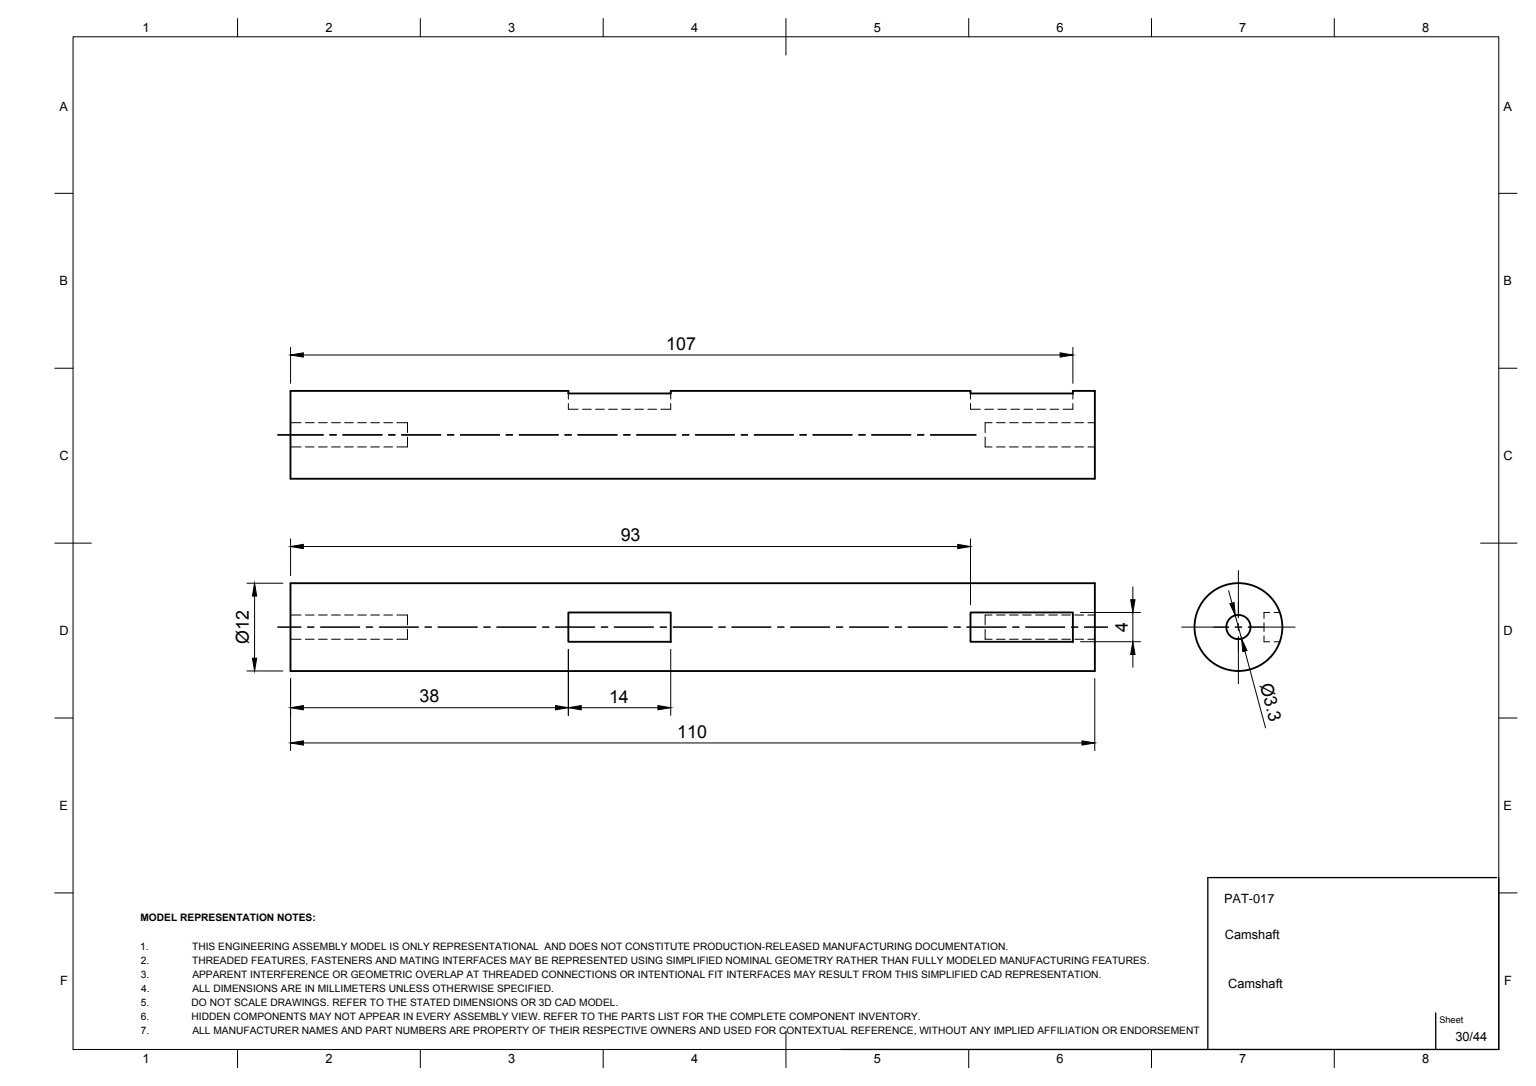
ISO-10303-21;
HEADER;
/* Generated by software containing ST-Developer
 * from STEP Tools, Inc. (www.steptools.com) 
 */

FILE_DESCRIPTION(
/* description */ ('Cam-and-follower valve demonstrator'),
/* implementation_level */ '2;1');

FILE_NAME(
/* name */ 'Camshaft.step',
/* time_stamp */ '2026-10-28T03:25:17-07:00',
/* author */ (''),
/* organization */ (''),
/* preprocessor_version */ 'ST-DEVELOPER v20.2',
/* originating_system */ 'Autodesk Translation Framework v15.17.0.0',
/* authorisation */ '');

FILE_SCHEMA (('AUTOMOTIVE_DESIGN { 1 0 10303 214 3 1 1 }'));
ENDSEC;

DATA;
#10=MECHANICAL_DESIGN_GEOMETRIC_PRESENTATION_REPRESENTATION('',(#440),#12896);
#361=SHAPE_REPRESENTATION_RELATIONSHIP('SRR','None',#13080,#397);
#397=ADVANCED_BREP_SHAPE_REPRESENTATION('',(#481),#12880);
#440=STYLED_ITEM('',(#13330),#481);
#481=MANIFOLD_SOLID_BREP('Body1',#6209);
#626=FACE_BOUND('',#1862,.T.);
#627=FACE_BOUND('',#1863,.T.);
#628=FACE_BOUND('',#1865,.T.);
#629=FACE_BOUND('',#1867,.T.);
#897=CIRCLE('',#7147,0.165);
#898=CIRCLE('',#7148,0.165);
#899=CIRCLE('',#7151,0.165);
#900=CIRCLE('',#7152,0.165);
#901=CIRCLE('',#7156,0.6);
#902=CIRCLE('',#7160,0.6);
#903=CIRCLE('',#7163,0.6);
#904=CIRCLE('',#7167,0.6);
#905=CIRCLE('',#7169,0.6);
#906=CIRCLE('',#7170,0.6);
#1062=CYLINDRICAL_SURFACE('',#7146,0.165);
#1063=CYLINDRICAL_SURFACE('',#7150,0.165);
#1064=CYLINDRICAL_SURFACE('',#7168,0.6);
#1348=FACE_OUTER_BOUND('',#1847,.T.);
#1349=FACE_OUTER_BOUND('',#1848,.T.);
#1350=FACE_OUTER_BOUND('',#1849,.T.);
#1351=FACE_OUTER_BOUND('',#1850,.T.);
#1352=FACE_OUTER_BOUND('',#1851,.T.);
#1353=FACE_OUTER_BOUND('',#1852,.T.);
#1354=FACE_OUTER_BOUND('',#1853,.T.);
#1355=FACE_OUTER_BOUND('',#1854,.T.);
#1356=FACE_OUTER_BOUND('',#1855,.T.);
#1357=FACE_OUTER_BOUND('',#1856,.T.);
#1358=FACE_OUTER_BOUND('',#1857,.T.);
#1359=FACE_OUTER_BOUND('',#1858,.T.);
#1360=FACE_OUTER_BOUND('',#1859,.T.);
#1361=FACE_OUTER_BOUND('',#1860,.T.);
#1362=FACE_OUTER_BOUND('',#1861,.T.);
#1363=FACE_OUTER_BOUND('',#1864,.T.);
#1364=FACE_OUTER_BOUND('',#1866,.T.);
#1847=EDGE_LOOP('',(#5173,#5174,#5175,#5176));
#1848=EDGE_LOOP('',(#5177));
#1849=EDGE_LOOP('',(#5178,#5179,#5180,#5181));
#1850=EDGE_LOOP('',(#5182));
#1851=EDGE_LOOP('',(#5183,#5184,#5185,#5186));
#1852=EDGE_LOOP('',(#5187,#5188,#5189,#5190));
#1853=EDGE_LOOP('',(#5191,#5192,#5193,#5194));
#1854=EDGE_LOOP('',(#5195,#5196,#5197,#5198));
#1855=EDGE_LOOP('',(#5199,#5200,#5201,#5202));
#1856=EDGE_LOOP('',(#5203,#5204,#5205,#5206));
#1857=EDGE_LOOP('',(#5207,#5208,#5209,#5210));
#1858=EDGE_LOOP('',(#5211,#5212,#5213,#5214));
#1859=EDGE_LOOP('',(#5215,#5216,#5217,#5218));
#1860=EDGE_LOOP('',(#5219,#5220,#5221,#5222));
#1861=EDGE_LOOP('',(#5223,#5224,#5225,#5226));
#1862=EDGE_LOOP('',(#5227,#5228,#5229,#5230));
#1863=EDGE_LOOP('',(#5231,#5232,#5233,#5234));
#1864=EDGE_LOOP('',(#5235));
#1865=EDGE_LOOP('',(#5236));
#1866=EDGE_LOOP('',(#5237));
#1867=EDGE_LOOP('',(#5238));
#2281=LINE('',#12271,#2703);
#2282=LINE('',#12278,#2704);
#2283=LINE('',#12284,#2705);
#2284=LINE('',#12286,#2706);
#2285=LINE('',#12288,#2707);
#2286=LINE('',#12289,#2708);
#2287=LINE('',#12294,#2709);
#2288=LINE('',#12295,#2710);
#2289=LINE('',#12298,#2711);
#2290=LINE('',#12300,#2712);
#2291=LINE('',#12301,#2713);
#2292=LINE('',#12303,#2714);
#2293=LINE('',#12309,#2715);
#2294=LINE('',#12311,#2716);
#2295=LINE('',#12313,#2717);
#2296=LINE('',#12314,#2718);
#2297=LINE('',#12319,#2719);
#2298=LINE('',#12320,#2720);
#2299=LINE('',#12323,#2721);
#2300=LINE('',#12325,#2722);
#2301=LINE('',#12326,#2723);
#2302=LINE('',#12328,#2724);
#2303=LINE('',#12335,#2725);
#2703=VECTOR('',#8752,0.165);
#2704=VECTOR('',#8761,0.165);
#2705=VECTOR('',#8768,1.);
#2706=VECTOR('',#8769,1.);
#2707=VECTOR('',#8770,1.);
#2708=VECTOR('',#8771,1.);
#2709=VECTOR('',#8776,1.);
#2710=VECTOR('',#8777,1.);
#2711=VECTOR('',#8780,1.);
#2712=VECTOR('',#8781,1.);
#2713=VECTOR('',#8782,1.);
#2714=VECTOR('',#8785,1.);
#2715=VECTOR('',#8792,1.);
#2716=VECTOR('',#8793,1.);
#2717=VECTOR('',#8794,1.);
#2718=VECTOR('',#8795,1.);
#2719=VECTOR('',#8800,1.);
#2720=VECTOR('',#8801,1.);
#2721=VECTOR('',#8804,1.);
#2722=VECTOR('',#8805,1.);
#2723=VECTOR('',#8806,1.);
#2724=VECTOR('',#8809,1.);
#2725=VECTOR('',#8818,0.6);
#3204=VERTEX_POINT('',#12268);
#3205=VERTEX_POINT('',#12270);
#3206=VERTEX_POINT('',#12275);
#3207=VERTEX_POINT('',#12277);
#3208=VERTEX_POINT('',#12282);
#3209=VERTEX_POINT('',#12283);
#3210=VERTEX_POINT('',#12285);
#3211=VERTEX_POINT('',#12287);
#3212=VERTEX_POINT('',#12291);
#3213=VERTEX_POINT('',#12293);
#3214=VERTEX_POINT('',#12297);
#3215=VERTEX_POINT('',#12299);
#3216=VERTEX_POINT('',#12307);
#3217=VERTEX_POINT('',#12308);
#3218=VERTEX_POINT('',#12310);
#3219=VERTEX_POINT('',#12312);
#3220=VERTEX_POINT('',#12316);
#3221=VERTEX_POINT('',#12318);
#3222=VERTEX_POINT('',#12322);
#3223=VERTEX_POINT('',#12324);
#3224=VERTEX_POINT('',#12332);
#3225=VERTEX_POINT('',#12334);
#3883=EDGE_CURVE('',#3204,#3204,#897,.T.);
#3884=EDGE_CURVE('',#3204,#3205,#2281,.T.);
#3885=EDGE_CURVE('',#3205,#3205,#898,.T.);
#3886=EDGE_CURVE('',#3206,#3206,#899,.T.);
#3887=EDGE_CURVE('',#3206,#3207,#2282,.T.);
#3888=EDGE_CURVE('',#3207,#3207,#900,.T.);
#3889=EDGE_CURVE('',#3208,#3209,#2283,.T.);
#3890=EDGE_CURVE('',#3208,#3210,#2284,.T.);
#3891=EDGE_CURVE('',#3211,#3210,#2285,.T.);
#3892=EDGE_CURVE('',#3211,#3209,#2286,.T.);
#3893=EDGE_CURVE('',#3209,#3212,#901,.T.);
#3894=EDGE_CURVE('',#3213,#3211,#2287,.T.);
#3895=EDGE_CURVE('',#3212,#3213,#2288,.T.);
#3896=EDGE_CURVE('',#3212,#3214,#2289,.T.);
#3897=EDGE_CURVE('',#3213,#3215,#2290,.T.);
#3898=EDGE_CURVE('',#3215,#3214,#2291,.T.);
#3899=EDGE_CURVE('',#3210,#3215,#2292,.T.);
#3900=EDGE_CURVE('',#3214,#3208,#902,.T.);
#3901=EDGE_CURVE('',#3216,#3217,#2293,.T.);
#3902=EDGE_CURVE('',#3216,#3218,#2294,.T.);
#3903=EDGE_CURVE('',#3219,#3218,#2295,.T.);
#3904=EDGE_CURVE('',#3219,#3217,#2296,.T.);
#3905=EDGE_CURVE('',#3217,#3220,#903,.T.);
#3906=EDGE_CURVE('',#3221,#3219,#2297,.T.);
#3907=EDGE_CURVE('',#3220,#3221,#2298,.T.);
#3908=EDGE_CURVE('',#3220,#3222,#2299,.T.);
#3909=EDGE_CURVE('',#3221,#3223,#2300,.T.);
#3910=EDGE_CURVE('',#3223,#3222,#2301,.T.);
#3911=EDGE_CURVE('',#3218,#3223,#2302,.T.);
#3912=EDGE_CURVE('',#3222,#3216,#904,.T.);
#3913=EDGE_CURVE('',#3224,#3224,#905,.T.);
#3914=EDGE_CURVE('',#3224,#3225,#2303,.T.);
#3915=EDGE_CURVE('',#3225,#3225,#906,.T.);
#5173=ORIENTED_EDGE('',*,*,#3883,.F.);
#5174=ORIENTED_EDGE('',*,*,#3884,.T.);
#5175=ORIENTED_EDGE('',*,*,#3885,.F.);
#5176=ORIENTED_EDGE('',*,*,#3884,.F.);
#5177=ORIENTED_EDGE('',*,*,#3883,.T.);
#5178=ORIENTED_EDGE('',*,*,#3886,.F.);
#5179=ORIENTED_EDGE('',*,*,#3887,.T.);
#5180=ORIENTED_EDGE('',*,*,#3888,.T.);
#5181=ORIENTED_EDGE('',*,*,#3887,.F.);
#5182=ORIENTED_EDGE('',*,*,#3888,.F.);
#5183=ORIENTED_EDGE('',*,*,#3889,.F.);
#5184=ORIENTED_EDGE('',*,*,#3890,.T.);
#5185=ORIENTED_EDGE('',*,*,#3891,.F.);
#5186=ORIENTED_EDGE('',*,*,#3892,.T.);
#5187=ORIENTED_EDGE('',*,*,#3893,.F.);
#5188=ORIENTED_EDGE('',*,*,#3892,.F.);
#5189=ORIENTED_EDGE('',*,*,#3894,.F.);
#5190=ORIENTED_EDGE('',*,*,#3895,.F.);
#5191=ORIENTED_EDGE('',*,*,#3896,.F.);
#5192=ORIENTED_EDGE('',*,*,#3895,.T.);
#5193=ORIENTED_EDGE('',*,*,#3897,.T.);
#5194=ORIENTED_EDGE('',*,*,#3898,.T.);
#5195=ORIENTED_EDGE('',*,*,#3894,.T.);
#5196=ORIENTED_EDGE('',*,*,#3891,.T.);
#5197=ORIENTED_EDGE('',*,*,#3899,.T.);
#5198=ORIENTED_EDGE('',*,*,#3897,.F.);
#5199=ORIENTED_EDGE('',*,*,#3900,.F.);
#5200=ORIENTED_EDGE('',*,*,#3898,.F.);
#5201=ORIENTED_EDGE('',*,*,#3899,.F.);
#5202=ORIENTED_EDGE('',*,*,#3890,.F.);
#5203=ORIENTED_EDGE('',*,*,#3901,.F.);
#5204=ORIENTED_EDGE('',*,*,#3902,.T.);
#5205=ORIENTED_EDGE('',*,*,#3903,.F.);
#5206=ORIENTED_EDGE('',*,*,#3904,.T.);
#5207=ORIENTED_EDGE('',*,*,#3905,.F.);
#5208=ORIENTED_EDGE('',*,*,#3904,.F.);
#5209=ORIENTED_EDGE('',*,*,#3906,.F.);
#5210=ORIENTED_EDGE('',*,*,#3907,.F.);
#5211=ORIENTED_EDGE('',*,*,#3908,.F.);
#5212=ORIENTED_EDGE('',*,*,#3907,.T.);
#5213=ORIENTED_EDGE('',*,*,#3909,.T.);
#5214=ORIENTED_EDGE('',*,*,#3910,.T.);
#5215=ORIENTED_EDGE('',*,*,#3906,.T.);
#5216=ORIENTED_EDGE('',*,*,#3903,.T.);
#5217=ORIENTED_EDGE('',*,*,#3911,.T.);
#5218=ORIENTED_EDGE('',*,*,#3909,.F.);
#5219=ORIENTED_EDGE('',*,*,#3912,.F.);
#5220=ORIENTED_EDGE('',*,*,#3910,.F.);
#5221=ORIENTED_EDGE('',*,*,#3911,.F.);
#5222=ORIENTED_EDGE('',*,*,#3902,.F.);
#5223=ORIENTED_EDGE('',*,*,#3913,.F.);
#5224=ORIENTED_EDGE('',*,*,#3914,.T.);
#5225=ORIENTED_EDGE('',*,*,#3915,.T.);
#5226=ORIENTED_EDGE('',*,*,#3914,.F.);
#5227=ORIENTED_EDGE('',*,*,#3896,.T.);
#5228=ORIENTED_EDGE('',*,*,#3900,.T.);
#5229=ORIENTED_EDGE('',*,*,#3889,.T.);
#5230=ORIENTED_EDGE('',*,*,#3893,.T.);
#5231=ORIENTED_EDGE('',*,*,#3908,.T.);
#5232=ORIENTED_EDGE('',*,*,#3912,.T.);
#5233=ORIENTED_EDGE('',*,*,#3901,.T.);
#5234=ORIENTED_EDGE('',*,*,#3905,.T.);
#5235=ORIENTED_EDGE('',*,*,#3913,.T.);
#5236=ORIENTED_EDGE('',*,*,#3885,.T.);
#5237=ORIENTED_EDGE('',*,*,#3915,.F.);
#5238=ORIENTED_EDGE('',*,*,#3886,.T.);
#5733=PLANE('',#7149);
#5734=PLANE('',#7153);
#5735=PLANE('',#7154);
#5736=PLANE('',#7155);
#5737=PLANE('',#7157);
#5738=PLANE('',#7158);
#5739=PLANE('',#7159);
#5740=PLANE('',#7161);
#5741=PLANE('',#7162);
#5742=PLANE('',#7164);
#5743=PLANE('',#7165);
#5744=PLANE('',#7166);
#5745=PLANE('',#7171);
#5746=PLANE('',#7172);
#6064=ADVANCED_FACE('',(#1348),#1062,.F.);
#6065=ADVANCED_FACE('',(#1349),#5733,.T.);
#6066=ADVANCED_FACE('',(#1350),#1063,.F.);
#6067=ADVANCED_FACE('',(#1351),#5734,.F.);
#6068=ADVANCED_FACE('',(#1352),#5735,.F.);
#6069=ADVANCED_FACE('',(#1353),#5736,.T.);
#6070=ADVANCED_FACE('',(#1354),#5737,.F.);
#6071=ADVANCED_FACE('',(#1355),#5738,.F.);
#6072=ADVANCED_FACE('',(#1356),#5739,.F.);
#6073=ADVANCED_FACE('',(#1357),#5740,.F.);
#6074=ADVANCED_FACE('',(#1358),#5741,.T.);
#6075=ADVANCED_FACE('',(#1359),#5742,.F.);
#6076=ADVANCED_FACE('',(#1360),#5743,.F.);
#6077=ADVANCED_FACE('',(#1361),#5744,.F.);
#6078=ADVANCED_FACE('',(#1362,#626,#627),#1064,.T.);
#6079=ADVANCED_FACE('',(#1363,#628),#5745,.T.);
#6080=ADVANCED_FACE('',(#1364,#629),#5746,.F.);
#6209=CLOSED_SHELL('',(#6064,#6065,#6066,#6067,#6068,#6069,#6070,#6071,
#6072,#6073,#6074,#6075,#6076,#6077,#6078,#6079,#6080));
#7145=AXIS2_PLACEMENT_3D('',#12266,#8746,#8747);
#7146=AXIS2_PLACEMENT_3D('',#12267,#8748,#8749);
#7147=AXIS2_PLACEMENT_3D('',#12269,#8750,#8751);
#7148=AXIS2_PLACEMENT_3D('',#12272,#8753,#8754);
#7149=AXIS2_PLACEMENT_3D('',#12273,#8755,#8756);
#7150=AXIS2_PLACEMENT_3D('',#12274,#8757,#8758);
#7151=AXIS2_PLACEMENT_3D('',#12276,#8759,#8760);
#7152=AXIS2_PLACEMENT_3D('',#12279,#8762,#8763);
#7153=AXIS2_PLACEMENT_3D('',#12280,#8764,#8765);
#7154=AXIS2_PLACEMENT_3D('',#12281,#8766,#8767);
#7155=AXIS2_PLACEMENT_3D('',#12290,#8772,#8773);
#7156=AXIS2_PLACEMENT_3D('',#12292,#8774,#8775);
#7157=AXIS2_PLACEMENT_3D('',#12296,#8778,#8779);
#7158=AXIS2_PLACEMENT_3D('',#12302,#8783,#8784);
#7159=AXIS2_PLACEMENT_3D('',#12304,#8786,#8787);
#7160=AXIS2_PLACEMENT_3D('',#12305,#8788,#8789);
#7161=AXIS2_PLACEMENT_3D('',#12306,#8790,#8791);
#7162=AXIS2_PLACEMENT_3D('',#12315,#8796,#8797);
#7163=AXIS2_PLACEMENT_3D('',#12317,#8798,#8799);
#7164=AXIS2_PLACEMENT_3D('',#12321,#8802,#8803);
#7165=AXIS2_PLACEMENT_3D('',#12327,#8807,#8808);
#7166=AXIS2_PLACEMENT_3D('',#12329,#8810,#8811);
#7167=AXIS2_PLACEMENT_3D('',#12330,#8812,#8813);
#7168=AXIS2_PLACEMENT_3D('',#12331,#8814,#8815);
#7169=AXIS2_PLACEMENT_3D('',#12333,#8816,#8817);
#7170=AXIS2_PLACEMENT_3D('',#12336,#8819,#8820);
#7171=AXIS2_PLACEMENT_3D('',#12337,#8821,#8822);
#7172=AXIS2_PLACEMENT_3D('',#12338,#8823,#8824);
#8746=DIRECTION('axis',(0.,0.,1.));
#8747=DIRECTION('refdir',(1.,0.,0.));
#8748=DIRECTION('center_axis',(0.,1.,0.));
#8749=DIRECTION('ref_axis',(1.,0.,0.));
#8750=DIRECTION('center_axis',(0.,1.,0.));
#8751=DIRECTION('ref_axis',(1.,0.,0.));
#8752=DIRECTION('',(0.,1.,0.));
#8753=DIRECTION('center_axis',(0.,-1.,0.));
#8754=DIRECTION('ref_axis',(1.,0.,0.));
#8755=DIRECTION('center_axis',(0.,1.,0.));
#8756=DIRECTION('ref_axis',(1.,0.,0.));
#8757=DIRECTION('center_axis',(0.,1.,0.));
#8758=DIRECTION('ref_axis',(1.,0.,0.));
#8759=DIRECTION('center_axis',(0.,1.,0.));
#8760=DIRECTION('ref_axis',(1.,0.,0.));
#8761=DIRECTION('',(0.,1.,0.));
#8762=DIRECTION('center_axis',(0.,1.,0.));
#8763=DIRECTION('ref_axis',(1.,0.,0.));
#8764=DIRECTION('center_axis',(0.,1.,0.));
#8765=DIRECTION('ref_axis',(1.,0.,0.));
#8766=DIRECTION('center_axis',(-1.,0.,0.));
#8767=DIRECTION('ref_axis',(0.,0.,1.));
#8768=DIRECTION('',(0.,-1.,0.));
#8769=DIRECTION('',(0.,0.,1.));
#8770=DIRECTION('',(0.,1.,0.));
#8771=DIRECTION('',(0.,0.,-1.));
#8772=DIRECTION('center_axis',(0.,1.,0.));
#8773=DIRECTION('ref_axis',(1.,0.,0.));
#8774=DIRECTION('center_axis',(0.,-1.,0.));
#8775=DIRECTION('ref_axis',(1.,0.,0.));
#8776=DIRECTION('',(-1.,0.,0.));
#8777=DIRECTION('',(0.,0.,1.));
#8778=DIRECTION('center_axis',(1.,0.,0.));
#8779=DIRECTION('ref_axis',(0.,0.,-1.));
#8780=DIRECTION('',(0.,1.,0.));
#8781=DIRECTION('',(0.,1.,0.));
#8782=DIRECTION('',(0.,0.,-1.));
#8783=DIRECTION('center_axis',(0.,0.,1.));
#8784=DIRECTION('ref_axis',(1.,0.,0.));
#8785=DIRECTION('',(1.,0.,0.));
#8786=DIRECTION('center_axis',(0.,1.,0.));
#8787=DIRECTION('ref_axis',(0.,0.,1.));
#8788=DIRECTION('center_axis',(0.,1.,0.));
#8789=DIRECTION('ref_axis',(1.,0.,0.));
#8790=DIRECTION('center_axis',(-1.,0.,0.));
#8791=DIRECTION('ref_axis',(0.,0.,1.));
#8792=DIRECTION('',(0.,-1.,0.));
#8793=DIRECTION('',(0.,0.,1.));
#8794=DIRECTION('',(0.,1.,0.));
#8795=DIRECTION('',(0.,0.,-1.));
#8796=DIRECTION('center_axis',(0.,1.,0.));
#8797=DIRECTION('ref_axis',(1.,0.,0.));
#8798=DIRECTION('center_axis',(0.,-1.,0.));
#8799=DIRECTION('ref_axis',(1.,0.,0.));
#8800=DIRECTION('',(-1.,0.,0.));
#8801=DIRECTION('',(0.,0.,1.));
#8802=DIRECTION('center_axis',(1.,0.,0.));
#8803=DIRECTION('ref_axis',(0.,0.,-1.));
#8804=DIRECTION('',(0.,1.,0.));
#8805=DIRECTION('',(0.,1.,0.));
#8806=DIRECTION('',(0.,0.,-1.));
#8807=DIRECTION('center_axis',(0.,0.,1.));
#8808=DIRECTION('ref_axis',(1.,0.,0.));
#8809=DIRECTION('',(1.,0.,0.));
#8810=DIRECTION('center_axis',(0.,1.,0.));
#8811=DIRECTION('ref_axis',(0.,0.,1.));
#8812=DIRECTION('center_axis',(0.,1.,0.));
#8813=DIRECTION('ref_axis',(1.,0.,0.));
#8814=DIRECTION('center_axis',(0.,1.,0.));
#8815=DIRECTION('ref_axis',(1.,0.,0.));
#8816=DIRECTION('center_axis',(0.,1.,0.));
#8817=DIRECTION('ref_axis',(1.,0.,0.));
#8818=DIRECTION('',(0.,-1.,0.));
#8819=DIRECTION('center_axis',(0.,1.,0.));
#8820=DIRECTION('ref_axis',(1.,0.,0.));
#8821=DIRECTION('center_axis',(0.,1.,0.));
#8822=DIRECTION('ref_axis',(1.,0.,0.));
#8823=DIRECTION('center_axis',(0.,1.,0.));
#8824=DIRECTION('ref_axis',(1.,0.,0.));
#12266=CARTESIAN_POINT('',(0.,0.,0.));
#12267=CARTESIAN_POINT('Origin',(0.,5.,4.));
#12268=CARTESIAN_POINT('',(-0.165,5.,4.));
#12269=CARTESIAN_POINT('Origin',(0.,5.,4.));
#12270=CARTESIAN_POINT('',(-0.165,6.5,4.));
#12271=CARTESIAN_POINT('',(-0.165,5.,4.));
#12272=CARTESIAN_POINT('Origin',(0.,6.5,4.));
#12273=CARTESIAN_POINT('Origin',(0.,5.,4.));
#12274=CARTESIAN_POINT('Origin',(0.,-4.6,4.));
#12275=CARTESIAN_POINT('',(-0.165,-4.5,4.));
#12276=CARTESIAN_POINT('Origin',(0.,-4.5,4.));
#12277=CARTESIAN_POINT('',(-0.165,-2.9,4.));
#12278=CARTESIAN_POINT('',(-0.165,-4.6,4.));
#12279=CARTESIAN_POINT('Origin',(0.,-2.9,4.));
#12280=CARTESIAN_POINT('Origin',(0.,-2.9,4.));
#12281=CARTESIAN_POINT('Origin',(-0.2,4.8,3.3));
#12282=CARTESIAN_POINT('',(-0.2,6.2,3.43431457505076));
#12283=CARTESIAN_POINT('',(-0.2,4.8,3.43431457505076));
#12284=CARTESIAN_POINT('',(-0.2,-4.5,3.43431457505076));
#12285=CARTESIAN_POINT('',(-0.2,6.2,3.65));
#12286=CARTESIAN_POINT('',(-0.2,6.2,3.65));
#12287=CARTESIAN_POINT('',(-0.2,4.8,3.65));
#12288=CARTESIAN_POINT('',(-0.2,4.8,3.65));
#12289=CARTESIAN_POINT('',(-0.2,4.8,3.65));
#12290=CARTESIAN_POINT('Origin',(0.,4.8,3.475));
#12291=CARTESIAN_POINT('',(0.2,4.8,3.43431457505076));
#12292=CARTESIAN_POINT('Origin',(0.,4.8,4.));
#12293=CARTESIAN_POINT('',(0.2,4.8,3.65));
#12294=CARTESIAN_POINT('',(0.2,4.8,3.65));
#12295=CARTESIAN_POINT('',(0.2,4.8,3.3));
#12296=CARTESIAN_POINT('Origin',(0.2,4.8,3.65));
#12297=CARTESIAN_POINT('',(0.2,6.2,3.43431457505076));
#12298=CARTESIAN_POINT('',(0.2,-4.5,3.43431457505076));
#12299=CARTESIAN_POINT('',(0.2,6.2,3.65));
#12300=CARTESIAN_POINT('',(0.2,4.8,3.65));
#12301=CARTESIAN_POINT('',(0.2,6.2,3.3));
#12302=CARTESIAN_POINT('Origin',(-0.2,4.8,3.65));
#12303=CARTESIAN_POINT('',(0.2,6.2,3.65));
#12304=CARTESIAN_POINT('Origin',(0.,6.2,3.475));
#12305=CARTESIAN_POINT('Origin',(0.,6.2,4.));
#12306=CARTESIAN_POINT('Origin',(-0.2,-0.7,3.3));
#12307=CARTESIAN_POINT('',(-0.2,0.7,3.43431457505076));
#12308=CARTESIAN_POINT('',(-0.2,-0.7,3.43431457505076));
#12309=CARTESIAN_POINT('',(-0.2,-4.5,3.43431457505076));
#12310=CARTESIAN_POINT('',(-0.2,0.7,3.65));
#12311=CARTESIAN_POINT('',(-0.2,0.7,3.65));
#12312=CARTESIAN_POINT('',(-0.2,-0.7,3.65));
#12313=CARTESIAN_POINT('',(-0.2,-0.7,3.65));
#12314=CARTESIAN_POINT('',(-0.2,-0.7,3.65));
#12315=CARTESIAN_POINT('Origin',(0.,-0.7,3.475));
#12316=CARTESIAN_POINT('',(0.2,-0.7,3.43431457505076));
#12317=CARTESIAN_POINT('Origin',(0.,-0.7,4.));
#12318=CARTESIAN_POINT('',(0.2,-0.7,3.65));
#12319=CARTESIAN_POINT('',(0.2,-0.7,3.65));
#12320=CARTESIAN_POINT('',(0.2,-0.7,3.3));
#12321=CARTESIAN_POINT('Origin',(0.2,-0.7,3.65));
#12322=CARTESIAN_POINT('',(0.2,0.7,3.43431457505076));
#12323=CARTESIAN_POINT('',(0.2,-4.5,3.43431457505076));
#12324=CARTESIAN_POINT('',(0.2,0.7,3.65));
#12325=CARTESIAN_POINT('',(0.2,-0.7,3.65));
#12326=CARTESIAN_POINT('',(0.2,0.7,3.3));
#12327=CARTESIAN_POINT('Origin',(-0.2,-0.7,3.65));
#12328=CARTESIAN_POINT('',(0.2,0.7,3.65));
#12329=CARTESIAN_POINT('Origin',(0.,0.7,3.475));
#12330=CARTESIAN_POINT('Origin',(0.,0.7,4.));
#12331=CARTESIAN_POINT('Origin',(0.,-4.5,4.));
#12332=CARTESIAN_POINT('',(-0.6,6.5,4.));
#12333=CARTESIAN_POINT('Origin',(0.,6.5,4.));
#12334=CARTESIAN_POINT('',(-0.6,-4.5,4.));
#12335=CARTESIAN_POINT('',(-0.6,-4.5,4.));
#12336=CARTESIAN_POINT('Origin',(0.,-4.5,4.));
#12337=CARTESIAN_POINT('Origin',(0.,6.5,4.));
#12338=CARTESIAN_POINT('Origin',(0.,-4.5,4.));
#12837=UNCERTAINTY_MEASURE_WITH_UNIT(LENGTH_MEASURE(0.001),#12897,
'DISTANCE_ACCURACY_VALUE',
'Maximum model space distance between geometric entities at asserted c
onnectivities');
#12853=UNCERTAINTY_MEASURE_WITH_UNIT(LENGTH_MEASURE(0.001),#12897,
'DISTANCE_ACCURACY_VALUE',
'Maximum model space distance between geometric entities at asserted c
onnectivities');
#12880=(
GEOMETRIC_REPRESENTATION_CONTEXT(3)
GLOBAL_UNCERTAINTY_ASSIGNED_CONTEXT((#12837))
GLOBAL_UNIT_ASSIGNED_CONTEXT((#12897,#12899,#12900))
REPRESENTATION_CONTEXT('','3D')
);
#12896=(
GEOMETRIC_REPRESENTATION_CONTEXT(3)
GLOBAL_UNCERTAINTY_ASSIGNED_CONTEXT((#12853))
GLOBAL_UNIT_ASSIGNED_CONTEXT((#12897,#12899,#12900))
REPRESENTATION_CONTEXT('','3D')
);
#12897=(
LENGTH_UNIT()
NAMED_UNIT(*)
SI_UNIT(.CENTI.,.METRE.)
);
#12899=(
NAMED_UNIT(*)
PLANE_ANGLE_UNIT()
SI_UNIT($,.RADIAN.)
);
#12900=(
NAMED_UNIT(*)
SI_UNIT($,.STERADIAN.)
SOLID_ANGLE_UNIT()
);
#12927=SHAPE_DEFINITION_REPRESENTATION(#12976,#13080);
#12976=PRODUCT_DEFINITION_SHAPE('',$,#13123);
#13080=SHAPE_REPRESENTATION('',(#7145),#12880);
#13096=PRODUCT_DEFINITION_CONTEXT('part definition',#13224,'design');
#13123=PRODUCT_DEFINITION('Camshaft','Camshaft',#13165,#13096);
#13165=PRODUCT_DEFINITION_FORMATION('',$,#13252);
#13224=APPLICATION_CONTEXT(
'Core Data for Automotive Mechanical Design Process');
#13225=PRODUCT_CONTEXT('part definition',#13224,'mechanical');
#13252=PRODUCT('Camshaft','Camshaft','Camshaft',(#13225));
#13324=COLOUR_RGB('Grey',0.48,0.52,0.57);
#13325=FILL_AREA_STYLE_COLOUR('',#13324);
#13326=FILL_AREA_STYLE('',(#13325));
#13327=SURFACE_STYLE_FILL_AREA(#13326);
#13328=SURFACE_SIDE_STYLE('',(#13327));
#13329=SURFACE_STYLE_USAGE(.BOTH.,#13328);
#13330=PRESENTATION_STYLE_ASSIGNMENT((#13329));
ENDSEC;
END-ISO-10303-21;
